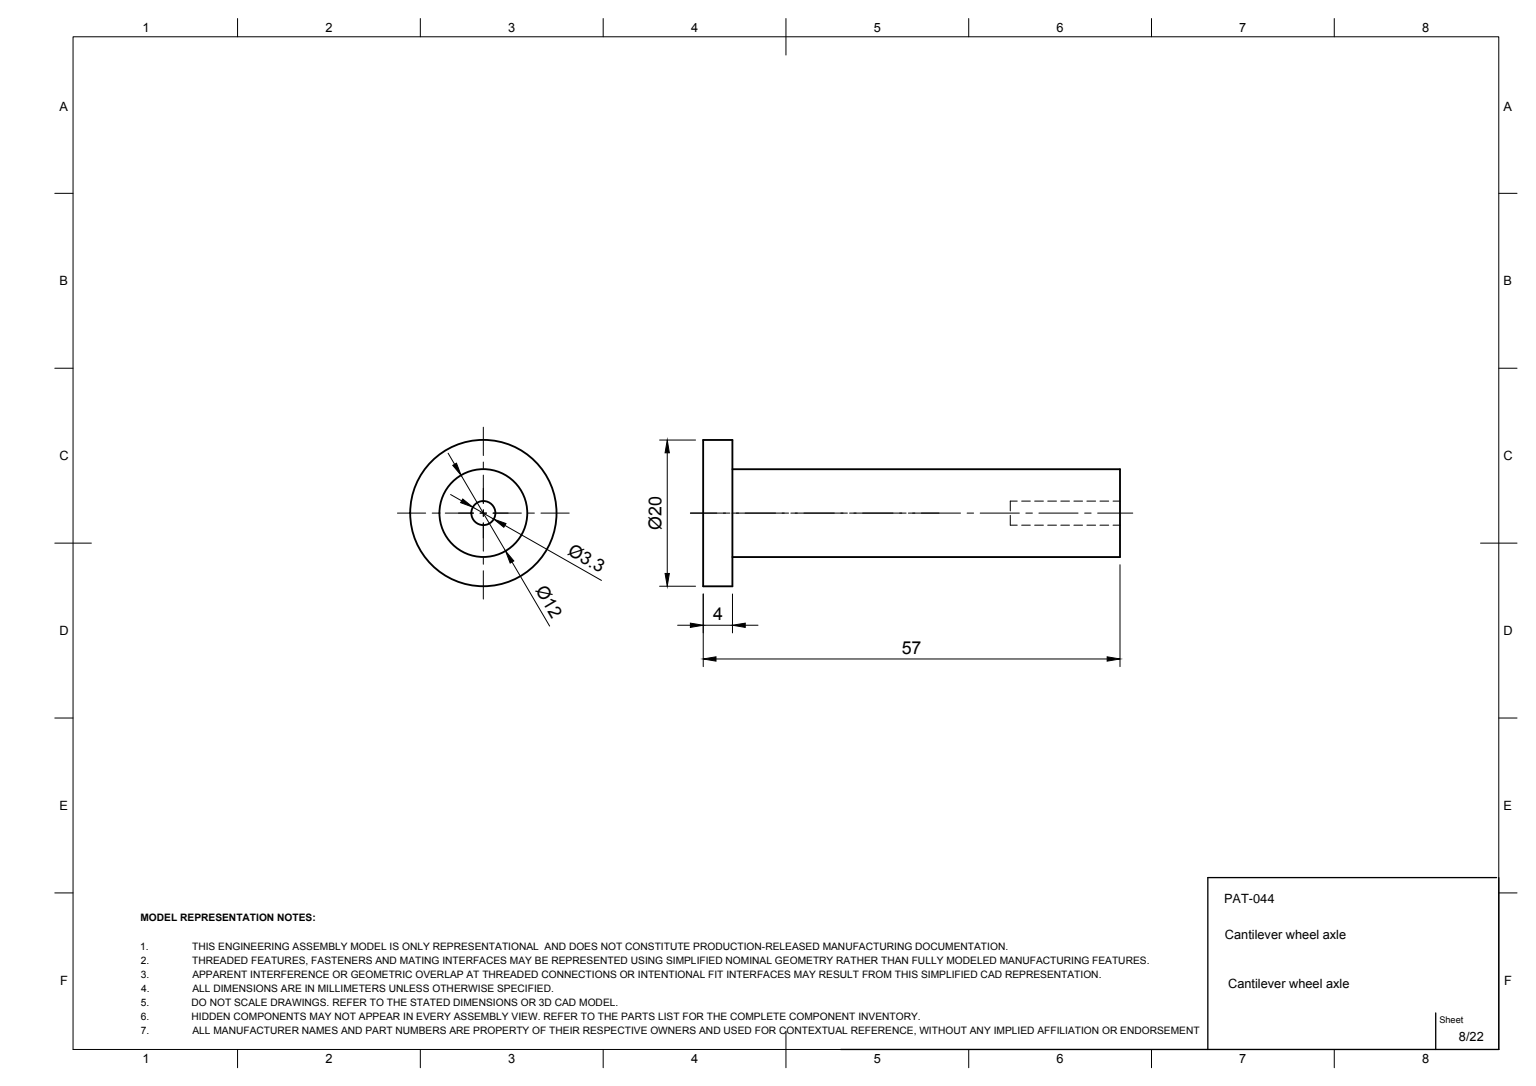
ISO-10303-21;
HEADER;
/* Generated by software containing ST-Developer
 * from STEP Tools, Inc. (www.steptools.com) 
 */

FILE_DESCRIPTION(
/* description */ ('Four-wheel beam trolley'),
/* implementation_level */ '2;1');

FILE_NAME(
/* name */ 'Cantilever wheel axle.step',
/* time_stamp */ '2026-10-29T16:22:06-07:00',
/* author */ (''),
/* organization */ (''),
/* preprocessor_version */ 'ST-DEVELOPER v20.2',
/* originating_system */ 'Autodesk Translation Framework v15.17.0.0',
/* authorisation */ '');

FILE_SCHEMA (('AUTOMOTIVE_DESIGN { 1 0 10303 214 3 1 1 }'));
ENDSEC;

DATA;
#10=MECHANICAL_DESIGN_GEOMETRIC_PRESENTATION_REPRESENTATION('',(#283),#4777);
#249=SHAPE_REPRESENTATION_RELATIONSHIP('SRR','None',#4878,#266);
#266=ADVANCED_BREP_SHAPE_REPRESENTATION('',(#306),#4763);
#283=STYLED_ITEM('',(#5056),#306);
#306=MANIFOLD_SOLID_BREP('Body1',#2371);
#341=FACE_BOUND('',#661,.T.);
#342=FACE_BOUND('',#666,.T.);
#399=PLANE('',#2674);
#400=PLANE('',#2675);
#401=PLANE('',#2680);
#402=PLANE('',#2683);
#494=FACE_OUTER_BOUND('',#658,.T.);
#495=FACE_OUTER_BOUND('',#659,.T.);
#496=FACE_OUTER_BOUND('',#660,.T.);
#497=FACE_OUTER_BOUND('',#662,.T.);
#498=FACE_OUTER_BOUND('',#663,.T.);
#499=FACE_OUTER_BOUND('',#664,.T.);
#500=FACE_OUTER_BOUND('',#665,.T.);
#658=EDGE_LOOP('',(#1827,#1828,#1829,#1830));
#659=EDGE_LOOP('',(#1831));
#660=EDGE_LOOP('',(#1832));
#661=EDGE_LOOP('',(#1833));
#662=EDGE_LOOP('',(#1834,#1835,#1836,#1837));
#663=EDGE_LOOP('',(#1838));
#664=EDGE_LOOP('',(#1839,#1840,#1841,#1842));
#665=EDGE_LOOP('',(#1843));
#666=EDGE_LOOP('',(#1844));
#846=LINE('',#3992,#969);
#847=LINE('',#4003,#970);
#848=LINE('',#4007,#971);
#969=VECTOR('',#3189,0.165);
#970=VECTOR('',#3204,1.);
#971=VECTOR('',#3209,0.6);
#1055=CIRCLE('',#2672,0.165);
#1056=CIRCLE('',#2673,0.165);
#1057=CIRCLE('',#2676,1.);
#1058=CIRCLE('',#2677,0.6);
#1059=CIRCLE('',#2679,1.);
#1060=CIRCLE('',#2682,0.6);
#1227=VERTEX_POINT('',#3989);
#1228=VERTEX_POINT('',#3991);
#1229=VERTEX_POINT('',#3996);
#1230=VERTEX_POINT('',#3998);
#1231=VERTEX_POINT('',#4001);
#1232=VERTEX_POINT('',#4006);
#1451=EDGE_CURVE('',#1227,#1227,#1055,.T.);
#1452=EDGE_CURVE('',#1227,#1228,#846,.T.);
#1453=EDGE_CURVE('',#1228,#1228,#1056,.T.);
#1454=EDGE_CURVE('',#1229,#1229,#1057,.T.);
#1455=EDGE_CURVE('',#1230,#1230,#1058,.T.);
#1456=EDGE_CURVE('',#1231,#1231,#1059,.T.);
#1457=EDGE_CURVE('',#1231,#1229,#847,.T.);
#1458=EDGE_CURVE('',#1230,#1232,#848,.T.);
#1459=EDGE_CURVE('',#1232,#1232,#1060,.T.);
#1827=ORIENTED_EDGE('',*,*,#1451,.F.);
#1828=ORIENTED_EDGE('',*,*,#1452,.T.);
#1829=ORIENTED_EDGE('',*,*,#1453,.T.);
#1830=ORIENTED_EDGE('',*,*,#1452,.F.);
#1831=ORIENTED_EDGE('',*,*,#1453,.F.);
#1832=ORIENTED_EDGE('',*,*,#1454,.F.);
#1833=ORIENTED_EDGE('',*,*,#1455,.T.);
#1834=ORIENTED_EDGE('',*,*,#1456,.F.);
#1835=ORIENTED_EDGE('',*,*,#1457,.T.);
#1836=ORIENTED_EDGE('',*,*,#1454,.T.);
#1837=ORIENTED_EDGE('',*,*,#1457,.F.);
#1838=ORIENTED_EDGE('',*,*,#1456,.T.);
#1839=ORIENTED_EDGE('',*,*,#1455,.F.);
#1840=ORIENTED_EDGE('',*,*,#1458,.T.);
#1841=ORIENTED_EDGE('',*,*,#1459,.T.);
#1842=ORIENTED_EDGE('',*,*,#1458,.F.);
#1843=ORIENTED_EDGE('',*,*,#1459,.F.);
#1844=ORIENTED_EDGE('',*,*,#1451,.T.);
#2189=CYLINDRICAL_SURFACE('',#2671,0.165);
#2190=CYLINDRICAL_SURFACE('',#2678,1.);
#2191=CYLINDRICAL_SURFACE('',#2681,0.6);
#2270=ADVANCED_FACE('',(#494),#2189,.F.);
#2271=ADVANCED_FACE('',(#495),#399,.F.);
#2272=ADVANCED_FACE('',(#496,#341),#400,.F.);
#2273=ADVANCED_FACE('',(#497),#2190,.T.);
#2274=ADVANCED_FACE('',(#498),#401,.T.);
#2275=ADVANCED_FACE('',(#499),#2191,.T.);
#2276=ADVANCED_FACE('',(#500,#342),#402,.F.);
#2371=CLOSED_SHELL('',(#2270,#2271,#2272,#2273,#2274,#2275,#2276));
#2670=AXIS2_PLACEMENT_3D('',#3987,#3183,#3184);
#2671=AXIS2_PLACEMENT_3D('',#3988,#3185,#3186);
#2672=AXIS2_PLACEMENT_3D('',#3990,#3187,#3188);
#2673=AXIS2_PLACEMENT_3D('',#3993,#3190,#3191);
#2674=AXIS2_PLACEMENT_3D('',#3994,#3192,#3193);
#2675=AXIS2_PLACEMENT_3D('',#3995,#3194,#3195);
#2676=AXIS2_PLACEMENT_3D('',#3997,#3196,#3197);
#2677=AXIS2_PLACEMENT_3D('',#3999,#3198,#3199);
#2678=AXIS2_PLACEMENT_3D('',#4000,#3200,#3201);
#2679=AXIS2_PLACEMENT_3D('',#4002,#3202,#3203);
#2680=AXIS2_PLACEMENT_3D('',#4004,#3205,#3206);
#2681=AXIS2_PLACEMENT_3D('',#4005,#3207,#3208);
#2682=AXIS2_PLACEMENT_3D('',#4008,#3210,#3211);
#2683=AXIS2_PLACEMENT_3D('',#4009,#3212,#3213);
#3183=DIRECTION('axis',(0.,0.,1.));
#3184=DIRECTION('refdir',(1.,0.,0.));
#3185=DIRECTION('center_axis',(0.,1.,0.));
#3186=DIRECTION('ref_axis',(1.,0.,0.));
#3187=DIRECTION('center_axis',(0.,1.,0.));
#3188=DIRECTION('ref_axis',(1.,0.,0.));
#3189=DIRECTION('',(0.,1.,0.));
#3190=DIRECTION('center_axis',(0.,1.,0.));
#3191=DIRECTION('ref_axis',(1.,0.,0.));
#3192=DIRECTION('center_axis',(0.,1.,0.));
#3193=DIRECTION('ref_axis',(1.,0.,0.));
#3194=DIRECTION('center_axis',(0.,1.,0.));
#3195=DIRECTION('ref_axis',(1.,0.,0.));
#3196=DIRECTION('center_axis',(0.,1.,0.));
#3197=DIRECTION('ref_axis',(1.,0.,0.));
#3198=DIRECTION('center_axis',(0.,1.,0.));
#3199=DIRECTION('ref_axis',(1.,0.,0.));
#3200=DIRECTION('center_axis',(0.,1.,0.));
#3201=DIRECTION('ref_axis',(1.,0.,0.));
#3202=DIRECTION('center_axis',(0.,1.,0.));
#3203=DIRECTION('ref_axis',(1.,0.,0.));
#3204=DIRECTION('',(0.,-1.,0.));
#3205=DIRECTION('center_axis',(0.,1.,0.));
#3206=DIRECTION('ref_axis',(1.,0.,0.));
#3207=DIRECTION('center_axis',(0.,1.,0.));
#3208=DIRECTION('ref_axis',(1.,0.,0.));
#3209=DIRECTION('',(0.,-1.,0.));
#3210=DIRECTION('center_axis',(0.,1.,0.));
#3211=DIRECTION('ref_axis',(1.,0.,0.));
#3212=DIRECTION('center_axis',(0.,1.,0.));
#3213=DIRECTION('ref_axis',(1.,0.,0.));
#3987=CARTESIAN_POINT('',(0.,0.,0.));
#3988=CARTESIAN_POINT('Origin',(0.,0.9,13.75));
#3989=CARTESIAN_POINT('',(-0.165,1.,13.75));
#3990=CARTESIAN_POINT('Origin',(0.,1.,13.75));
#3991=CARTESIAN_POINT('',(-0.165,2.5,13.75));
#3992=CARTESIAN_POINT('',(-0.165,0.9,13.75));
#3993=CARTESIAN_POINT('Origin',(0.,2.5,13.75));
#3994=CARTESIAN_POINT('Origin',(0.,2.5,13.75));
#3995=CARTESIAN_POINT('Origin',(0.,6.3,13.75));
#3996=CARTESIAN_POINT('',(-1.,6.3,13.75));
#3997=CARTESIAN_POINT('Origin',(0.,6.3,13.75));
#3998=CARTESIAN_POINT('',(-0.6,6.3,13.75));
#3999=CARTESIAN_POINT('Origin',(0.,6.3,13.75));
#4000=CARTESIAN_POINT('Origin',(0.,6.3,13.75));
#4001=CARTESIAN_POINT('',(-1.,6.7,13.75));
#4002=CARTESIAN_POINT('Origin',(0.,6.7,13.75));
#4003=CARTESIAN_POINT('',(-1.,6.3,13.75));
#4004=CARTESIAN_POINT('Origin',(0.,6.7,13.75));
#4005=CARTESIAN_POINT('Origin',(0.,1.,13.75));
#4006=CARTESIAN_POINT('',(-0.6,1.,13.75));
#4007=CARTESIAN_POINT('',(-0.6,1.,13.75));
#4008=CARTESIAN_POINT('Origin',(0.,1.,13.75));
#4009=CARTESIAN_POINT('Origin',(0.,1.,13.75));
#4741=UNCERTAINTY_MEASURE_WITH_UNIT(LENGTH_MEASURE(0.001),#4778,
'DISTANCE_ACCURACY_VALUE',
'Maximum model space distance between geometric entities at asserted c
onnectivities');
#4755=UNCERTAINTY_MEASURE_WITH_UNIT(LENGTH_MEASURE(0.001),#4778,
'DISTANCE_ACCURACY_VALUE',
'Maximum model space distance between geometric entities at asserted c
onnectivities');
#4763=(
GEOMETRIC_REPRESENTATION_CONTEXT(3)
GLOBAL_UNCERTAINTY_ASSIGNED_CONTEXT((#4741))
GLOBAL_UNIT_ASSIGNED_CONTEXT((#4778,#4780,#4781))
REPRESENTATION_CONTEXT('','3D')
);
#4777=(
GEOMETRIC_REPRESENTATION_CONTEXT(3)
GLOBAL_UNCERTAINTY_ASSIGNED_CONTEXT((#4755))
GLOBAL_UNIT_ASSIGNED_CONTEXT((#4778,#4780,#4781))
REPRESENTATION_CONTEXT('','3D')
);
#4778=(
LENGTH_UNIT()
NAMED_UNIT(*)
SI_UNIT(.CENTI.,.METRE.)
);
#4780=(
NAMED_UNIT(*)
PLANE_ANGLE_UNIT()
SI_UNIT($,.RADIAN.)
);
#4781=(
NAMED_UNIT(*)
SI_UNIT($,.STERADIAN.)
SOLID_ANGLE_UNIT()
);
#4789=SHAPE_DEFINITION_REPRESENTATION(#4810,#4878);
#4810=PRODUCT_DEFINITION_SHAPE('',$,#4900);
#4878=SHAPE_REPRESENTATION('',(#2670),#4763);
#4892=PRODUCT_DEFINITION_CONTEXT('part definition',#4957,'design');
#4900=PRODUCT_DEFINITION('Cantilever wheel axle',
'Cantilever wheel axle',#4921,#4892);
#4921=PRODUCT_DEFINITION_FORMATION('',$,#4966);
#4957=APPLICATION_CONTEXT(
'Core Data for Automotive Mechanical Design Process');
#4958=PRODUCT_CONTEXT('part definition',#4957,'mechanical');
#4966=PRODUCT('Cantilever wheel axle','Cantilever wheel axle',
'Cantilever wheel axle',(#4958));
#5050=COLOUR_RGB('Grey',0.48,0.52,0.57);
#5051=FILL_AREA_STYLE_COLOUR('',#5050);
#5052=FILL_AREA_STYLE('',(#5051));
#5053=SURFACE_STYLE_FILL_AREA(#5052);
#5054=SURFACE_SIDE_STYLE('',(#5053));
#5055=SURFACE_STYLE_USAGE(.BOTH.,#5054);
#5056=PRESENTATION_STYLE_ASSIGNMENT((#5055));
ENDSEC;
END-ISO-10303-21;
